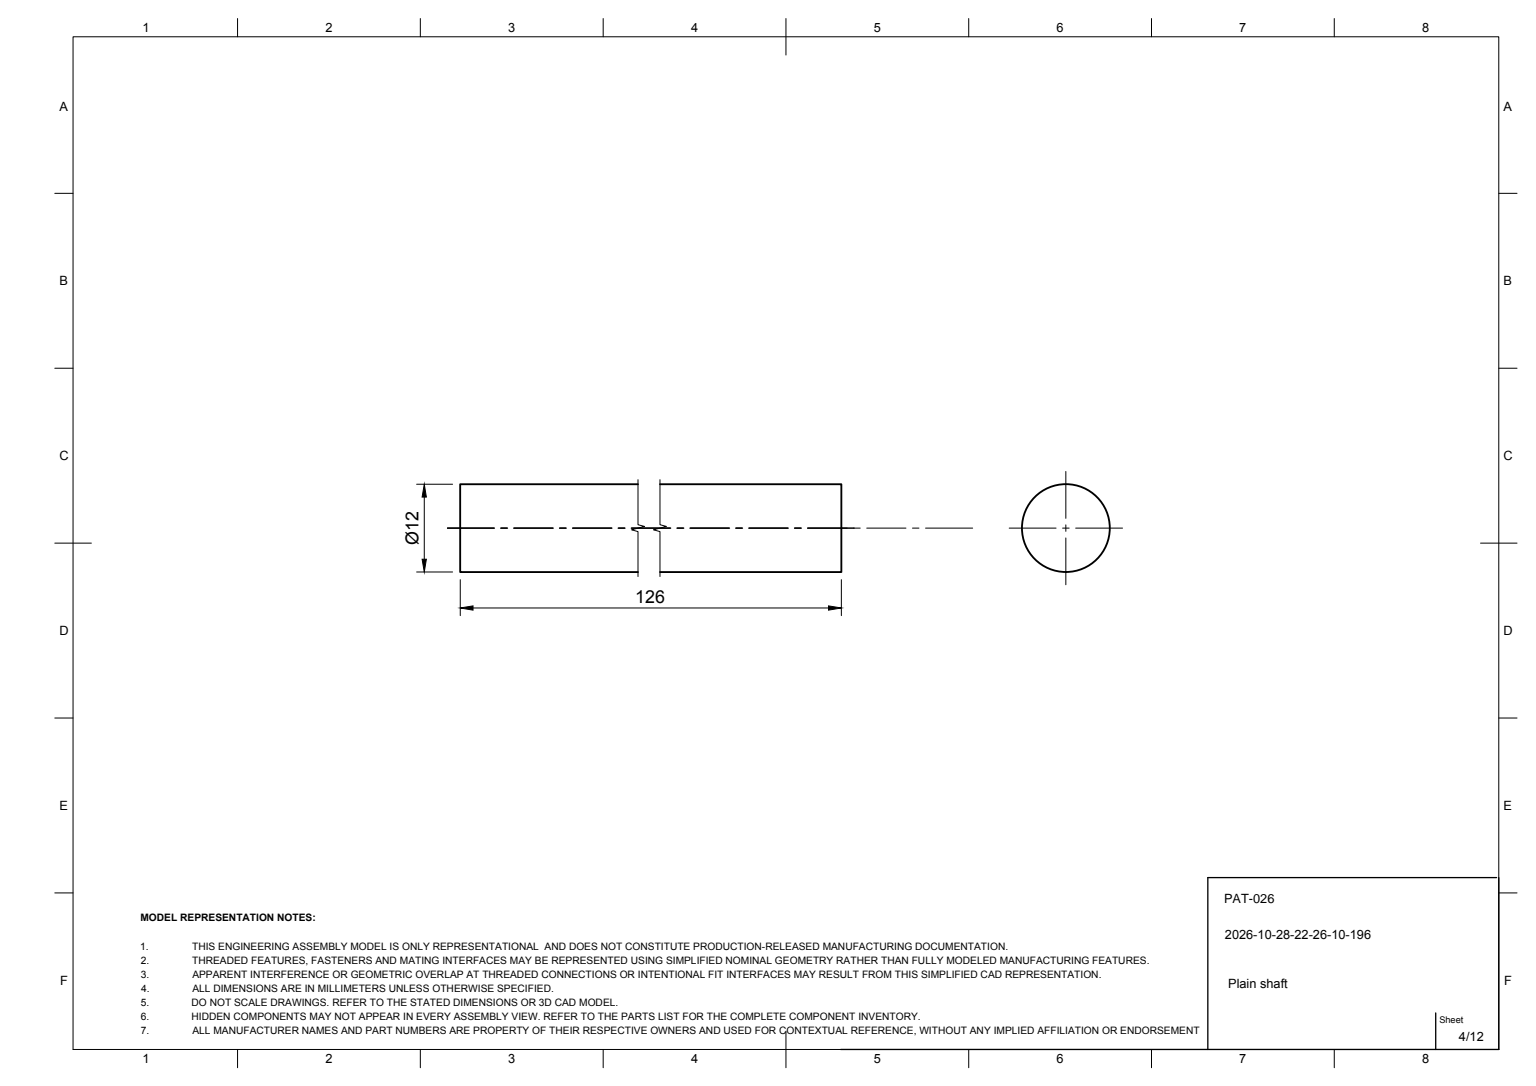
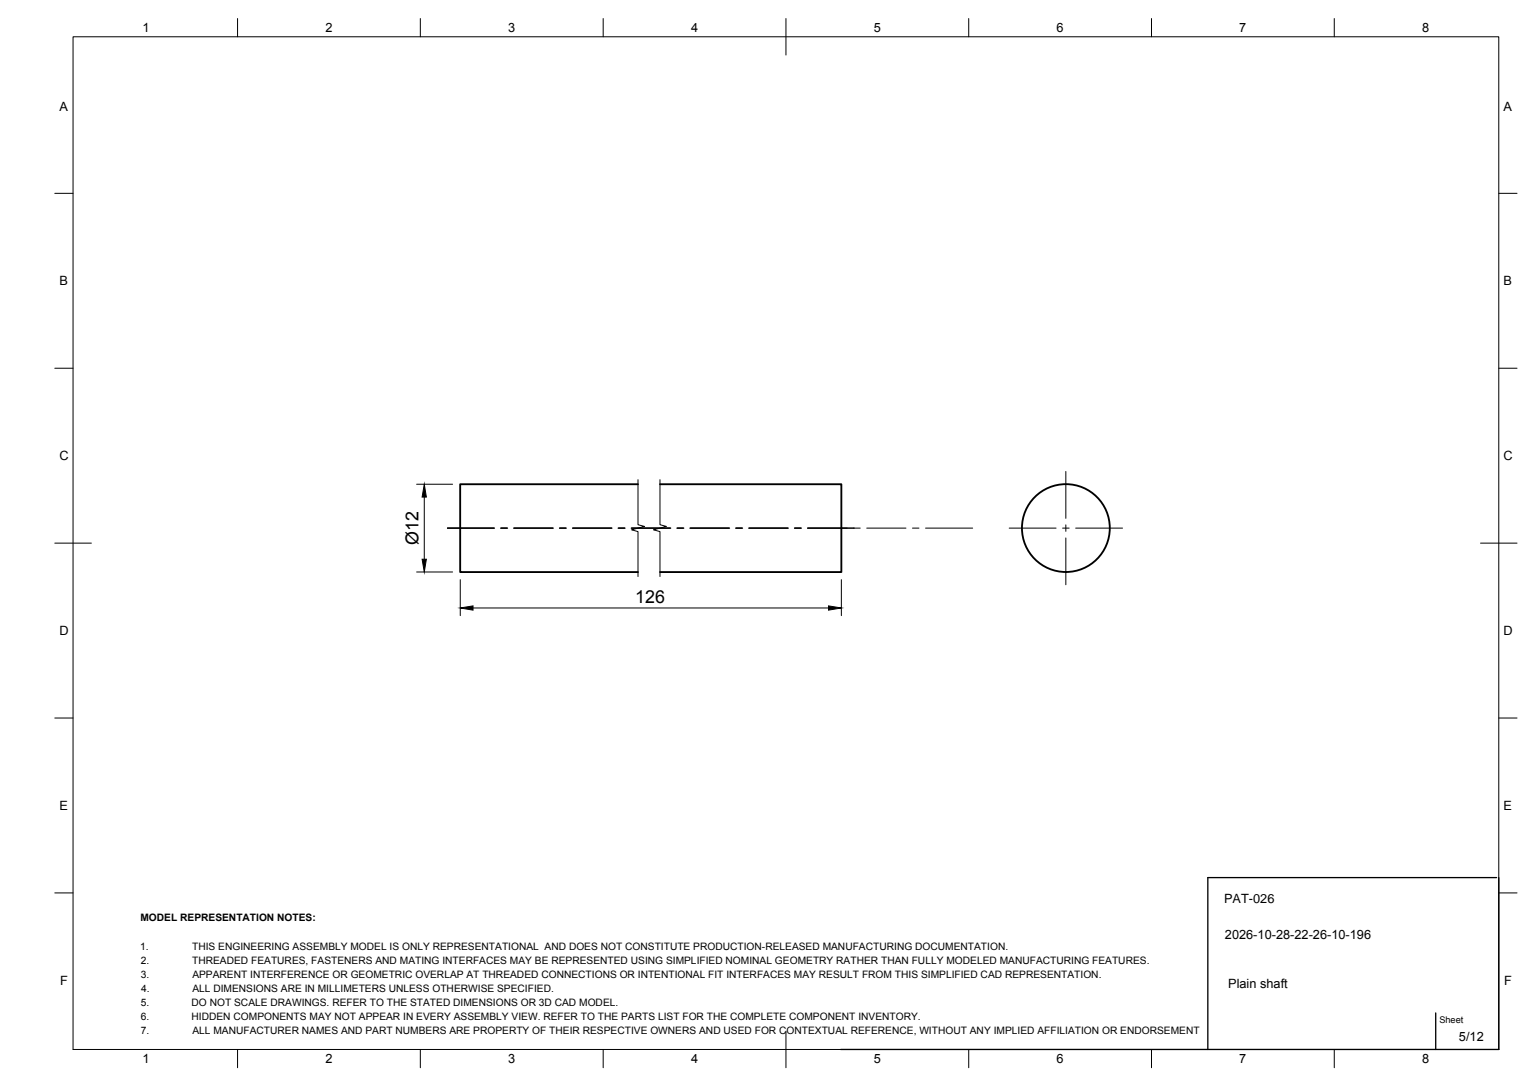
ISO-10303-21;
HEADER;
/* Generated by software containing ST-Developer
 * from STEP Tools, Inc. (www.steptools.com) 
 */

FILE_DESCRIPTION(
/* description */ ('PAT-026'),
/* implementation_level */ '2;1');

FILE_NAME(
/* name */ 'Plain shaft.step',
/* time_stamp */ '2026-10-28T22:25:58-07:00',
/* author */ (''),
/* organization */ (''),
/* preprocessor_version */ 'ST-DEVELOPER v20.2',
/* originating_system */ 'Autodesk Translation Framework v15.17.0.0',
/* authorisation */ '');

FILE_SCHEMA (('AUTOMOTIVE_DESIGN { 1 0 10303 214 3 1 1 }'));
ENDSEC;

DATA;
#10=MECHANICAL_DESIGN_GEOMETRIC_PRESENTATION_REPRESENTATION('',(#142),#12343);
#120=SHAPE_REPRESENTATION_RELATIONSHIP('SRR','None',#12397,#131);
#131=ADVANCED_BREP_SHAPE_REPRESENTATION('',(#153),#12332);
#142=STYLED_ITEM('',(#12533),#153);
#153=MANIFOLD_SOLID_BREP('Body1',#7348);
#200=PLANE('',#7506);
#201=PLANE('',#7507);
#563=FACE_OUTER_BOUND('',#974,.T.);
#564=FACE_OUTER_BOUND('',#975,.T.);
#565=FACE_OUTER_BOUND('',#976,.T.);
#974=EDGE_LOOP('',(#4947,#4948,#4949,#4950));
#975=EDGE_LOOP('',(#4951));
#976=EDGE_LOOP('',(#4952));
#1408=LINE('',#10097,#2280);
#2280=VECTOR('',#8106,0.6);
#3144=CIRCLE('',#7504,0.6);
#3145=CIRCLE('',#7505,0.6);
#3277=VERTEX_POINT('',#10094);
#3278=VERTEX_POINT('',#10096);
#3917=EDGE_CURVE('',#3277,#3277,#3144,.T.);
#3918=EDGE_CURVE('',#3277,#3278,#1408,.T.);
#3919=EDGE_CURVE('',#3278,#3278,#3145,.T.);
#4947=ORIENTED_EDGE('',*,*,#3917,.F.);
#4948=ORIENTED_EDGE('',*,*,#3918,.T.);
#4949=ORIENTED_EDGE('',*,*,#3919,.T.);
#4950=ORIENTED_EDGE('',*,*,#3918,.F.);
#4951=ORIENTED_EDGE('',*,*,#3917,.T.);
#4952=ORIENTED_EDGE('',*,*,#3919,.F.);
#6915=CYLINDRICAL_SURFACE('',#7503,0.6);
#6954=ADVANCED_FACE('',(#563),#6915,.T.);
#6955=ADVANCED_FACE('',(#564),#200,.T.);
#6956=ADVANCED_FACE('',(#565),#201,.F.);
#7348=CLOSED_SHELL('',(#6954,#6955,#6956));
#7502=AXIS2_PLACEMENT_3D('',#10092,#8100,#8101);
#7503=AXIS2_PLACEMENT_3D('',#10093,#8102,#8103);
#7504=AXIS2_PLACEMENT_3D('',#10095,#8104,#8105);
#7505=AXIS2_PLACEMENT_3D('',#10098,#8107,#8108);
#7506=AXIS2_PLACEMENT_3D('',#10099,#8109,#8110);
#7507=AXIS2_PLACEMENT_3D('',#10100,#8111,#8112);
#8100=DIRECTION('axis',(0.,0.,1.));
#8101=DIRECTION('refdir',(1.,0.,0.));
#8102=DIRECTION('center_axis',(0.,1.,0.));
#8103=DIRECTION('ref_axis',(1.,0.,0.));
#8104=DIRECTION('center_axis',(0.,1.,0.));
#8105=DIRECTION('ref_axis',(1.,0.,0.));
#8106=DIRECTION('',(0.,-1.,0.));
#8107=DIRECTION('center_axis',(0.,1.,0.));
#8108=DIRECTION('ref_axis',(1.,0.,0.));
#8109=DIRECTION('center_axis',(0.,1.,0.));
#8110=DIRECTION('ref_axis',(1.,0.,0.));
#8111=DIRECTION('center_axis',(0.,1.,0.));
#8112=DIRECTION('ref_axis',(1.,0.,0.));
#10092=CARTESIAN_POINT('',(0.,0.,0.));
#10093=CARTESIAN_POINT('Origin',(0.,-13.,3.5));
#10094=CARTESIAN_POINT('',(-0.6,-0.399999999999999,3.5));
#10095=CARTESIAN_POINT('Origin',(0.,-0.399999999999999,3.5));
#10096=CARTESIAN_POINT('',(-0.6,-13.,3.5));
#10097=CARTESIAN_POINT('',(-0.6,-13.,3.5));
#10098=CARTESIAN_POINT('Origin',(0.,-13.,3.5));
#10099=CARTESIAN_POINT('Origin',(0.,-0.399999999999999,3.5));
#10100=CARTESIAN_POINT('Origin',(0.,-13.,3.5));
#12318=UNCERTAINTY_MEASURE_WITH_UNIT(LENGTH_MEASURE(0.001),#12344,
'DISTANCE_ACCURACY_VALUE',
'Maximum model space distance between geometric entities at asserted c
onnectivities');
#12329=UNCERTAINTY_MEASURE_WITH_UNIT(LENGTH_MEASURE(0.001),#12344,
'DISTANCE_ACCURACY_VALUE',
'Maximum model space distance between geometric entities at asserted c
onnectivities');
#12332=(
GEOMETRIC_REPRESENTATION_CONTEXT(3)
GLOBAL_UNCERTAINTY_ASSIGNED_CONTEXT((#12318))
GLOBAL_UNIT_ASSIGNED_CONTEXT((#12344,#12346,#12347))
REPRESENTATION_CONTEXT('','3D')
);
#12343=(
GEOMETRIC_REPRESENTATION_CONTEXT(3)
GLOBAL_UNCERTAINTY_ASSIGNED_CONTEXT((#12329))
GLOBAL_UNIT_ASSIGNED_CONTEXT((#12344,#12346,#12347))
REPRESENTATION_CONTEXT('','3D')
);
#12344=(
LENGTH_UNIT()
NAMED_UNIT(*)
SI_UNIT(.CENTI.,.METRE.)
);
#12346=(
NAMED_UNIT(*)
PLANE_ANGLE_UNIT()
SI_UNIT($,.RADIAN.)
);
#12347=(
NAMED_UNIT(*)
SI_UNIT($,.STERADIAN.)
SOLID_ANGLE_UNIT()
);
#12350=SHAPE_DEFINITION_REPRESENTATION(#12363,#12397);
#12363=PRODUCT_DEFINITION_SHAPE('',$,#12411);
#12397=SHAPE_REPRESENTATION('',(#7502),#12332);
#12408=PRODUCT_DEFINITION_CONTEXT('part definition',#12449,'design');
#12411=PRODUCT_DEFINITION('Plain shaft','Plain shaft',#12424,
#12408);
#12424=PRODUCT_DEFINITION_FORMATION('',$,#12453);
#12449=APPLICATION_CONTEXT(
'Core Data for Automotive Mechanical Design Process');
#12450=PRODUCT_CONTEXT('part definition',#12449,'mechanical');
#12453=PRODUCT('Plain shaft','Plain shaft','Plain shaft',(#12450));
#12527=COLOUR_RGB('Grey',0.48,0.52,0.57);
#12528=FILL_AREA_STYLE_COLOUR('',#12527);
#12529=FILL_AREA_STYLE('',(#12528));
#12530=SURFACE_STYLE_FILL_AREA(#12529);
#12531=SURFACE_SIDE_STYLE('',(#12530));
#12532=SURFACE_STYLE_USAGE(.BOTH.,#12531);
#12533=PRESENTATION_STYLE_ASSIGNMENT((#12532));
ENDSEC;
END-ISO-10303-21;
